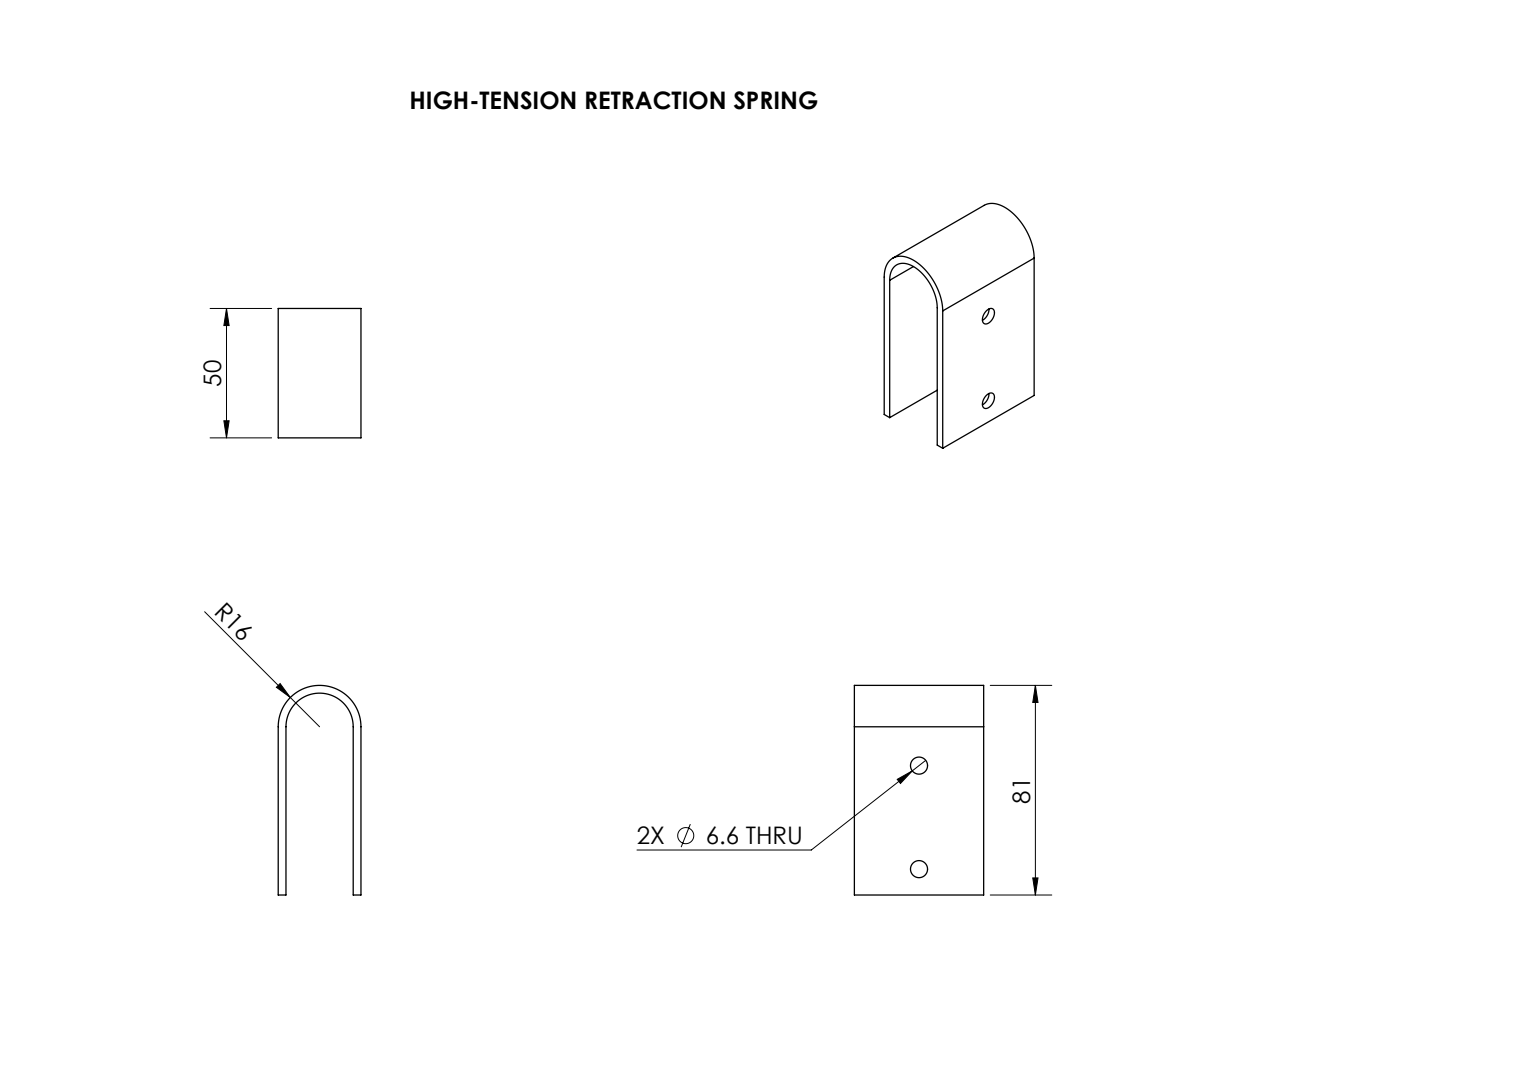
ISO-10303-21;
HEADER;
FILE_DESCRIPTION (('STEP AP214'),
    '1' );
FILE_NAME ('High-Tension Retraction Spring.step',
    '2026-09-24T10:26:00',
    ( '' ),
    ( '' ),
    'SwSTEP 2.0',
    'SolidWorks 2026',
    '' );
FILE_SCHEMA (( 'AUTOMOTIVE_DESIGN' ));
ENDSEC;

DATA;
#71=MECHANICAL_DESIGN_GEOMETRIC_PRESENTATION_REPRESENTATION('',(#7530),#1232);
#73=VERTEX_POINT ( 'NONE', #1987 ) ;
#74=AXIS2_PLACEMENT_3D ( 'NONE', #8274, #12524, #8346 ) ;
#146=ORIENTED_EDGE ( 'NONE', *, *, #7792, .F. ) ;
#147=EDGE_LOOP ( 'NONE', ( #10800, #705, #1394, #14407 ) ) ;
#167=CARTESIAN_POINT ( 'NONE',  ( 0.000000000000000000, 0.000000000000000000, 0.000000000000000000 ) ) ;
#344=ORIENTED_EDGE ( 'NONE', *, *, #679, .T. ) ;
#371=LINE ( 'NONE', #6940, #6098 ) ;
#406=EDGE_LOOP ( 'NONE', ( #12305, #13878, #13303, #2200 ) ) ;
#471=( LENGTH_UNIT ( ) NAMED_UNIT ( * ) SI_UNIT ( .MILLI., .METRE. ) );
#524=VECTOR ( 'NONE', #14360, 1000.000000000000000 ) ;
#530=FACE_BOUND ( 'NONE', #4280, .T. ) ;
#548=PRESENTATION_STYLE_ASSIGNMENT (( #10489 ) ) ;
#575=CARTESIAN_POINT ( 'NONE',  ( 79.68170757442804586, 124.5765550933606249, 25.00000000000000000 ) ) ;
#595=CARTESIAN_POINT ( 'NONE',  ( 79.68170757442804586, 59.57655509336061073, -25.00000000000000000 ) ) ;
#604=ORIENTED_EDGE ( 'NONE', *, *, #5491, .T. ) ;
#619=VERTEX_POINT ( 'NONE', #10072 ) ;
#629=( NAMED_UNIT ( * ) SI_UNIT ( $, .STERADIAN. ) SOLID_ANGLE_UNIT ( ) );
#656=AXIS2_PLACEMENT_3D ( 'NONE', #5018, #7273, #14033 ) ;
#679=EDGE_CURVE ( 'NONE', #13538, #9142, #13956, .T. ) ;
#688=CARTESIAN_POINT ( 'NONE',  ( 92.68170757442806007, 124.5765550933605965, 25.00000000000000000 ) ) ;
#704=VECTOR ( 'NONE', #1188, 1000.000000000000000 ) ;
#705=ORIENTED_EDGE ( 'NONE', *, *, #5491, .F. ) ;
#713=AXIS2_PLACEMENT_3D ( 'NONE', #14232, #7612, #6386 ) ;
#745=CARTESIAN_POINT ( 'NONE',  ( 105.6817075744281311, 124.5765550933606107, 25.00000000000000000 ) ) ;
#749=VECTOR ( 'NONE', #1705, 1000.000000000000000 ) ;
#843=CARTESIAN_POINT ( 'NONE',  ( 76.68170757442798902, 124.5765550933606249, 25.00000000000000000 ) ) ;
#858=DIRECTION ( 'NONE',  ( 1.000000000000000000, 0.000000000000000000, 0.000000000000000000 ) ) ;
#868=EDGE_CURVE ( 'NONE', #3118, #5760, #13014, .T. ) ;
#872=AXIS2_PLACEMENT_3D ( 'NONE', #10007, #2111, #11927 ) ;
#906=DIRECTION ( 'NONE',  ( 0.000000000000000000, 1.000000000000000000, 0.000000000000000000 ) ) ;
#907=CARTESIAN_POINT ( 'NONE',  ( 108.6817075744280174, 69.57655509336049704, 3.300000000000013589 ) ) ;
#929=LINE ( 'NONE', #7732, #11392 ) ;
#970=EDGE_LOOP ( 'NONE', ( #14106, #13551, #3898, #10691 ) ) ;
#985=LINE ( 'NONE', #843, #7180 ) ;
#1177=CIRCLE ( 'NONE', #713, 3.299999999999997158 ) ;
#1188=DIRECTION ( 'NONE',  ( -1.000000000000000000, 0.000000000000000000, 0.000000000000000000 ) ) ;
#1232=( GEOMETRIC_REPRESENTATION_CONTEXT ( 3 ) GLOBAL_UNCERTAINTY_ASSIGNED_CONTEXT ( ( #9384 ) ) GLOBAL_UNIT_ASSIGNED_CONTEXT ( ( #471, #8358, #629 ) ) REPRESENTATION_CONTEXT ( 'NONE', 'WORKASPACE' ) );
#1243=DIRECTION ( 'NONE',  ( -1.000000000000000000, 0.000000000000000000, 0.000000000000000000 ) ) ;
#1298=DIRECTION ( 'NONE',  ( 1.000000000000000000, 0.000000000000000000, 0.000000000000000000 ) ) ;
#1373=AXIS2_PLACEMENT_3D ( 'NONE', #5187, #4969, #7375 ) ;
#1393=VERTEX_POINT ( 'NONE', #9403 ) ;
#1394=ORIENTED_EDGE ( 'NONE', *, *, #679, .F. ) ;
#1475=LINE ( 'NONE', #2572, #5846 ) ;
#1487=ORIENTED_EDGE ( 'NONE', *, *, #12210, .T. ) ;
#1492=CARTESIAN_POINT ( 'NONE',  ( 108.6817075744280174, 109.5765550933605113, 1.102182119232617753E-14 ) ) ;
#1518=FILL_AREA_STYLE ('',( #12707 ) ) ;
#1556=CYLINDRICAL_SURFACE ( 'NONE', #13817, 3.299999999999997158 ) ;
#1558=( NAMED_UNIT ( * ) SI_UNIT ( $, .STERADIAN. ) SOLID_ANGLE_UNIT ( ) );
#1560=DIRECTION ( 'NONE',  ( 0.000000000000000000, 0.000000000000000000, 1.000000000000000000 ) ) ;
#1599=AXIS2_PLACEMENT_3D ( 'NONE', #5171, #7423, #11909 ) ;
#1606=EDGE_CURVE ( 'NONE', #1393, #8011, #1475, .T. ) ;
#1681=DIRECTION ( 'NONE',  ( 0.000000000000000000, 0.000000000000000000, -1.000000000000000000 ) ) ;
#1704=LINE ( 'NONE', #14151, #10227 ) ;
#1705=DIRECTION ( 'NONE',  ( 2.133709875451472726E-16, -1.000000000000000000, -0.000000000000000000 ) ) ;
#1708=VECTOR ( 'NONE', #2266, 1000.000000000000000 ) ;
#1717=SURFACE_STYLE_FILL_AREA ( #13940 ) ;
#1721=AXIS2_PLACEMENT_3D ( 'NONE', #688, #4065, #2281 ) ;
#1773=DIRECTION ( 'NONE',  ( -1.000000000000000000, 0.000000000000000000, 0.000000000000000000 ) ) ;
#1798=LINE ( 'NONE', #11825, #7044 ) ;
#1807=EDGE_LOOP ( 'NONE', ( #11288, #9763, #3211, #9884 ) ) ;
#1871=ADVANCED_FACE ( 'NONE', ( #12299 ), #3099, .F. ) ;
#1888=AXIS2_PLACEMENT_3D ( 'NONE', #7294, #2996, #12863 ) ;
#1979=FACE_OUTER_BOUND ( 'NONE', #5149, .T. ) ;
#1987=CARTESIAN_POINT ( 'NONE',  ( 79.68170757442804586, 59.57655509336061073, 25.00000000000000000 ) ) ;
#1996=LINE ( 'NONE', #12988, #749 ) ;
#2030=EDGE_CURVE ( 'NONE', #619, #2684, #5361, .T. ) ;
#2043=CIRCLE ( 'NONE', #7627, 3.299999999999997158 ) ;
#2050=ORIENTED_EDGE ( 'NONE', *, *, #4383, .F. ) ;
#2111=DIRECTION ( 'NONE',  ( 0.000000000000000000, -1.000000000000000000, 0.000000000000000000 ) ) ;
#2114=DIRECTION ( 'NONE',  ( 0.000000000000000000, 0.000000000000000000, -1.000000000000000000 ) ) ;
#2200=ORIENTED_EDGE ( 'NONE', *, *, #5207, .T. ) ;
#2266=DIRECTION ( 'NONE',  ( 0.000000000000000000, 0.000000000000000000, -1.000000000000000000 ) ) ;
#2281=DIRECTION ( 'NONE',  ( -1.000000000000000000, 0.000000000000000000, 0.000000000000000000 ) ) ;
#2305=PLANE ( 'NONE',  #12341 ) ;
#2311=EDGE_CURVE ( 'NONE', #5760, #13538, #5795, .T. ) ;
#2340=CARTESIAN_POINT ( 'NONE',  ( 92.68170757442806007, 124.5765550933605965, 25.00000000000000000 ) ) ;
#2344=CARTESIAN_POINT ( 'NONE',  ( 108.6817075744280174, 69.57655509336049704, -3.299999999999981171 ) ) ;
#2414=DIRECTION ( 'NONE',  ( -1.000000000000000000, 0.000000000000000000, 0.000000000000000000 ) ) ;
#2515=EDGE_CURVE ( 'NONE', #4441, #2985, #8459, .T. ) ;
#2528=ADVANCED_FACE ( 'NONE', ( #6107 ), #5028, .F. ) ;
#2572=CARTESIAN_POINT ( 'NONE',  ( 76.68170757442798902, 124.5765550933606249, -25.00000000000000000 ) ) ;
#2596=CARTESIAN_POINT ( 'NONE',  ( 108.6817075744280174, 109.5765550933605113, 1.102182119232617753E-14 ) ) ;
#2616=SURFACE_SIDE_STYLE ('',( #5960 ) ) ;
#2636=CARTESIAN_POINT ( 'NONE',  ( 108.6817075744280174, 69.57655509336049704, 1.592040838891559450E-14 ) ) ;
#2650=VECTOR ( 'NONE', #13343, 1000.000000000000000 ) ;
#2684=VERTEX_POINT ( 'NONE', #3272 ) ;
#2701=EDGE_CURVE ( 'NONE', #11645, #2779, #7907, .T. ) ;
#2723=EDGE_CURVE ( 'NONE', #11645, #12380, #9019, .T. ) ;
#2746=CARTESIAN_POINT ( 'NONE',  ( 92.68170757442806007, 124.5765550933605965, 25.00000000000000000 ) ) ;
#2755=DIRECTION ( 'NONE',  ( 1.000000000000000000, 0.000000000000000000, 0.000000000000000000 ) ) ;
#2771=CARTESIAN_POINT ( 'NONE',  ( 105.6817075744280174, 109.5765550933605113, -3.299999999999986500 ) ) ;
#2779=VERTEX_POINT ( 'NONE', #5522 ) ;
#2839=CARTESIAN_POINT ( 'NONE',  ( 76.68170757442798902, 124.5765550933606249, 25.00000000000000000 ) ) ;
#2862=LINE ( 'NONE', #12874, #11439 ) ;
#2912=FACE_OUTER_BOUND ( 'NONE', #9549, .T. ) ;
#2979=DIRECTION ( 'NONE',  ( 0.000000000000000000, 0.000000000000000000, -1.000000000000000000 ) ) ;
#2985=VERTEX_POINT ( 'NONE', #4346 ) ;
#2996=DIRECTION ( 'NONE',  ( 1.000000000000000000, 0.000000000000000000, 0.000000000000000000 ) ) ;
#3003=VERTEX_POINT ( 'NONE', #12232 ) ;
#3020=ORIENTED_EDGE ( 'NONE', *, *, #11613, .T. ) ;
#3022=CARTESIAN_POINT ( 'NONE',  ( 108.6817075744280174, 69.57655509336049704, 3.300000000000013589 ) ) ;
#3071=( GEOMETRIC_REPRESENTATION_CONTEXT ( 3 ) GLOBAL_UNCERTAINTY_ASSIGNED_CONTEXT ( ( #3983 ) ) GLOBAL_UNIT_ASSIGNED_CONTEXT ( ( #11535, #10370, #9264 ) ) REPRESENTATION_CONTEXT ( 'NONE', 'WORKASPACE' ) );
#3090=CARTESIAN_POINT ( 'NONE',  ( 108.6817075744280174, 109.5765550933605113, -3.299999999999986500 ) ) ;
#3096=ORIENTED_EDGE ( 'NONE', *, *, #7792, .T. ) ;
#3099=CYLINDRICAL_SURFACE ( 'NONE', #10041, 3.299999999999997158 ) ;
#3118=VERTEX_POINT ( 'NONE', #5219 ) ;
#3211=ORIENTED_EDGE ( 'NONE', *, *, #868, .F. ) ;
#3214=CARTESIAN_POINT ( 'NONE',  ( 92.68170757442806007, 124.5765550933605965, 25.00000000000000000 ) ) ;
#3253=LINE ( 'NONE', #9903, #5813 ) ;
#3272=CARTESIAN_POINT ( 'NONE',  ( 105.6817075744280174, 69.57655509336049704, -3.299999999999981171 ) ) ;
#3348=DIRECTION ( 'NONE',  ( 0.000000000000000000, -1.000000000000000000, 0.000000000000000000 ) ) ;
#3373=CARTESIAN_POINT ( 'NONE',  ( 108.6817075744280174, 109.5765550933605113, 3.300000000000008260 ) ) ;
#3449=CYLINDRICAL_SURFACE ( 'NONE', #6558, 13.00000000000002487 ) ;
#3453=AXIS2_PLACEMENT_3D ( 'NONE', #9492, #3717, #7286 ) ;
#3528=ORIENTED_EDGE ( 'NONE', *, *, #6801, .T. ) ;
#3559=FACE_OUTER_BOUND ( 'NONE', #406, .T. ) ;
#3597=LINE ( 'NONE', #10235, #4268 ) ;
#3601=EDGE_CURVE ( 'NONE', #619, #13436, #9629, .T. ) ;
#3628=CARTESIAN_POINT ( 'NONE',  ( 108.6817075744280174, 109.5765550933605113, -3.299999999999986500 ) ) ;
#3717=DIRECTION ( 'NONE',  ( 1.000000000000000000, 2.133709875451472726E-16, 0.000000000000000000 ) ) ;
#3736=DIRECTION ( 'NONE',  ( 1.000000000000000000, 0.000000000000000000, 0.000000000000000000 ) ) ;
#3766=DIRECTION ( 'NONE',  ( 1.000000000000000000, 0.000000000000000000, 0.000000000000000000 ) ) ;
#3863=DIRECTION ( 'NONE',  ( 2.133709875451472726E-16, -1.000000000000000000, -0.000000000000000000 ) ) ;
#3872=FACE_OUTER_BOUND ( 'NONE', #8424, .T. ) ;
#3881=DIRECTION ( 'NONE',  ( 0.000000000000000000, 0.000000000000000000, 1.000000000000000000 ) ) ;
#3898=ORIENTED_EDGE ( 'NONE', *, *, #9778, .T. ) ;
#3970=EDGE_CURVE ( 'NONE', #6982, #1393, #11344, .T. ) ;
#3983=UNCERTAINTY_MEASURE_WITH_UNIT (LENGTH_MEASURE( 1.000000000000000082E-05 ), #11535, 'distance_accuracy_value', 'NONE');
#4065=DIRECTION ( 'NONE',  ( 0.000000000000000000, 0.000000000000000000, -1.000000000000000000 ) ) ;
#4164=CARTESIAN_POINT ( 'NONE',  ( 108.6817075744280743, 124.5765550933606107, -25.00000000000000000 ) ) ;
#4252=CARTESIAN_POINT ( 'NONE',  ( 79.68170757442804586, 59.57655509336061073, -25.00000000000000000 ) ) ;
#4268=VECTOR ( 'NONE', #2414, 1000.000000000000000 ) ;
#4280=EDGE_LOOP ( 'NONE', ( #5320, #13667 ) ) ;
#4299=CARTESIAN_POINT ( 'NONE',  ( 108.6817075744280743, 59.57655509336061073, -25.00000000000000000 ) ) ;
#4302=ADVANCED_FACE ( 'NONE', ( #530, #10623, #11866 ), #8414, .T. ) ;
#4346=CARTESIAN_POINT ( 'NONE',  ( 105.6817075744281311, 124.5765550933606107, -25.00000000000000000 ) ) ;
#4371=ORIENTED_EDGE ( 'NONE', *, *, #9778, .F. ) ;
#4383=EDGE_CURVE ( 'NONE', #2684, #619, #4527, .T. ) ;
#4429=VECTOR ( 'NONE', #13663, 1000.000000000000000 ) ;
#4441=VERTEX_POINT ( 'NONE', #8845 ) ;
#4464=AXIS2_PLACEMENT_3D ( 'NONE', #13909, #3881, #8316 ) ;
#4490=LINE ( 'NONE', #2344, #524 ) ;
#4527=CIRCLE ( 'NONE', #9159, 3.299999999999997158 ) ;
#4530=CARTESIAN_POINT ( 'NONE',  ( 108.6817075744280743, 124.5765550933606107, -25.00000000000000000 ) ) ;
#4533=ORIENTED_EDGE ( 'NONE', *, *, #10521, .T. ) ;
#4559=FACE_OUTER_BOUND ( 'NONE', #970, .T. ) ;
#4770=VECTOR ( 'NONE', #3863, 1000.000000000000000 ) ;
#4792=DIRECTION ( 'NONE',  ( 0.000000000000000000, 0.000000000000000000, -1.000000000000000000 ) ) ;
#4847=EDGE_CURVE ( 'NONE', #13538, #1393, #985, .T. ) ;
#4879=CARTESIAN_POINT ( 'NONE',  ( 92.68170757442806007, 124.5765550933605965, -25.00000000000000000 ) ) ;
#4884=ORIENTED_EDGE ( 'NONE', *, *, #6439, .T. ) ;
#4901=ADVANCED_FACE ( 'NONE', ( #11302 ), #2305, .T. ) ;
#4913=DIRECTION ( 'NONE',  ( 0.000000000000000000, 1.000000000000000000, 0.000000000000000000 ) ) ;
#4950=CARTESIAN_POINT ( 'NONE',  ( 105.6817075744281311, 124.5765550933606107, -25.00000000000000000 ) ) ;
#4952=CARTESIAN_POINT ( 'NONE',  ( 105.6817075744281311, 124.5765550933606107, 25.00000000000000000 ) ) ;
#4954=AXIS2_PLACEMENT_3D ( 'NONE', #13901, #12782, #1298 ) ;
#4957=DIRECTION ( 'NONE',  ( 0.000000000000000000, 0.000000000000000000, 1.000000000000000000 ) ) ;
#4959=PLANE ( 'NONE',  #4954 ) ;
#4969=DIRECTION ( 'NONE',  ( -1.000000000000000000, 0.000000000000000000, 0.000000000000000000 ) ) ;
#4976=DIRECTION ( 'NONE',  ( 2.133709875451472726E-16, -1.000000000000000000, -0.000000000000000000 ) ) ;
#5018=CARTESIAN_POINT ( 'NONE',  ( 79.68170757442804586, 124.5765550933606249, 25.00000000000000000 ) ) ;
#5028=PLANE ( 'NONE',  #3453 ) ;
#5132=ORIENTED_EDGE ( 'NONE', *, *, #2515, .T. ) ;
#5138=EDGE_CURVE ( 'NONE', #3118, #14145, #6082, .T. ) ;
#5148=SHAPE_REPRESENTATION_RELATIONSHIP ( 'NONE' , 'NONE' ,  #10940, #5243 ) ;
#5149=EDGE_LOOP ( 'NONE', ( #13973, #11717, #6274, #14396 ) ) ;
#5156=ORIENTED_EDGE ( 'NONE', *, *, #1606, .F. ) ;
#5171=CARTESIAN_POINT ( 'NONE',  ( 105.6817075744280174, 109.5765550933605113, 1.102182119232617753E-14 ) ) ;
#5187=CARTESIAN_POINT ( 'NONE',  ( 105.6817075744280174, 69.57655509336051125, 1.592040838891559450E-14 ) ) ;
#5203=COLOUR_RGB ( '', 0.66274510, 0.83137255, 0.94901961) ;
#5207=EDGE_CURVE ( 'NONE', #12380, #11468, #1177, .T. ) ;
#5219=CARTESIAN_POINT ( 'NONE',  ( 108.6817075744280743, 59.57655509336061073, 25.00000000000000000 ) ) ;
#5243=ADVANCED_BREP_SHAPE_REPRESENTATION ( '', ( #11564, #11025 ), #7056 ) ;
#5273=EDGE_CURVE ( 'NONE', #2779, #11468, #3253, .T. ) ;
#5276=DIRECTION ( 'NONE',  ( -1.000000000000000000, 0.000000000000000000, 0.000000000000000000 ) ) ;
#5277=DIRECTION ( 'NONE',  ( 1.000000000000000000, 0.000000000000000000, 0.000000000000000000 ) ) ;
#5320=ORIENTED_EDGE ( 'NONE', *, *, #2701, .F. ) ;
#5361=CIRCLE ( 'NONE', #1373, 3.299999999999997158 ) ;
#5418=ADVANCED_FACE ( 'NONE', ( #6128 ), #8173, .F. ) ;
#5424=CARTESIAN_POINT ( 'NONE',  ( 79.68170757442804586, 59.57655509336061073, 25.00000000000000000 ) ) ;
#5441=DIRECTION ( 'NONE',  ( 1.000000000000000000, 0.000000000000000000, 0.000000000000000000 ) ) ;
#5491=EDGE_CURVE ( 'NONE', #9142, #8011, #2862, .T. ) ;
#5505=AXIS2_PLACEMENT_3D ( 'NONE', #7465, #10637, #6381 ) ;
#5522=CARTESIAN_POINT ( 'NONE',  ( 105.6817075744280174, 109.5765550933605113, 3.300000000000008260 ) ) ;
#5531=VERTEX_POINT ( 'NONE', #4252 ) ;
#5596=ORIENTED_EDGE ( 'NONE', *, *, #3970, .F. ) ;
#5760=VERTEX_POINT ( 'NONE', #10430 ) ;
#5795=CIRCLE ( 'NONE', #14021, 16.00000000000001421 ) ;
#5813=VECTOR ( 'NONE', #10988, 1000.000000000000000 ) ;
#5833=APPLICATION_CONTEXT ( 'automotive_design' ) ;
#5846=VECTOR ( 'NONE', #6884, 1000.000000000000000 ) ;
#5960=SURFACE_STYLE_FILL_AREA ( #1518 ) ;
#6024=ADVANCED_FACE ( 'NONE', ( #3559 ), #1556, .F. ) ;
#6036=SURFACE_STYLE_USAGE ( .BOTH. , #2616 ) ;
#6063=DIRECTION ( 'NONE',  ( 0.000000000000000000, 0.000000000000000000, 1.000000000000000000 ) ) ;
#6082=LINE ( 'NONE', #7109, #13045 ) ;
#6093=ORIENTED_EDGE ( 'NONE', *, *, #2701, .T. ) ;
#6098=VECTOR ( 'NONE', #4976, 1000.000000000000000 ) ;
#6107=FACE_OUTER_BOUND ( 'NONE', #147, .T. ) ;
#6108=LINE ( 'NONE', #4952, #13540 ) ;
#6128=FACE_OUTER_BOUND ( 'NONE', #6849, .T. ) ;
#6188=DIRECTION ( 'NONE',  ( 1.000000000000000000, 0.000000000000000000, 0.000000000000000000 ) ) ;
#6274=ORIENTED_EDGE ( 'NONE', *, *, #8411, .T. ) ;
#6281=PRODUCT_CONTEXT ( 'NONE', #5833, 'mechanical' ) ;
#6290=ORIENTED_EDGE ( 'NONE', *, *, #2515, .F. ) ;
#6292=CARTESIAN_POINT ( 'NONE',  ( 105.6817075744280174, 69.57655509336051125, 1.592040838891559450E-14 ) ) ;
#6372=ORIENTED_EDGE ( 'NONE', *, *, #13541, .F. ) ;
#6381=DIRECTION ( 'NONE',  ( 1.000000000000000000, 0.000000000000000000, 0.000000000000000000 ) ) ;
#6386=DIRECTION ( 'NONE',  ( 0.000000000000000000, 0.000000000000000000, -1.000000000000000000 ) ) ;
#6423=DIRECTION ( 'NONE',  ( 1.000000000000000000, 0.000000000000000000, 0.000000000000000000 ) ) ;
#6439=EDGE_CURVE ( 'NONE', #5531, #8011, #9354, .T. ) ;
#6452=ORIENTED_EDGE ( 'NONE', *, *, #12896, .T. ) ;
#6454=ADVANCED_FACE ( 'NONE', ( #10112 ), #9004, .F. ) ;
#6505=CIRCLE ( 'NONE', #12129, 3.299999999999997158 ) ;
#6524=DIRECTION ( 'NONE',  ( 0.000000000000000000, 0.000000000000000000, 1.000000000000000000 ) ) ;
#6558=AXIS2_PLACEMENT_3D ( 'NONE', #2340, #11267, #1243 ) ;
#6653=ORIENTED_EDGE ( 'NONE', *, *, #5207, .F. ) ;
#6766=EDGE_LOOP ( 'NONE', ( #6653, #9405 ) ) ;
#6783=CIRCLE ( 'NONE', #1888, 3.299999999999997158 ) ;
#6801=EDGE_CURVE ( 'NONE', #3003, #2985, #6108, .T. ) ;
#6829=PRODUCT_DEFINITION_SHAPE ( 'NONE', 'NONE',  #11417 ) ;
#6849=EDGE_LOOP ( 'NONE', ( #5156, #5596, #7420, #11471, #5132, #4533, #1487, #4884 ) ) ;
#6865=EDGE_CURVE ( 'NONE', #14145, #6982, #10665, .T. ) ;
#6884=DIRECTION ( 'NONE',  ( 2.133709875451472726E-16, -1.000000000000000000, -0.000000000000000000 ) ) ;
#6940=CARTESIAN_POINT ( 'NONE',  ( 79.68170757442804586, 124.5765550933606249, -25.00000000000000000 ) ) ;
#6959=VECTOR ( 'NONE', #9710, 1000.000000000000000 ) ;
#6982=VERTEX_POINT ( 'NONE', #4530 ) ;
#7044=VECTOR ( 'NONE', #2979, 1000.000000000000000 ) ;
#7056=( GEOMETRIC_REPRESENTATION_CONTEXT ( 3 ) GLOBAL_UNCERTAINTY_ASSIGNED_CONTEXT ( ( #9235 ) ) GLOBAL_UNIT_ASSIGNED_CONTEXT ( ( #11658, #9469, #1558 ) ) REPRESENTATION_CONTEXT ( 'NONE', 'WORKASPACE' ) );
#7062=PRESENTATION_STYLE_ASSIGNMENT (( #6036 ) ) ;
#7086=CARTESIAN_POINT ( 'NONE',  ( 105.6817075744280743, 59.57655509336061073, 25.00000000000000000 ) ) ;
#7091=VECTOR ( 'NONE', #906, 1000.000000000000000 ) ;
#7109=CARTESIAN_POINT ( 'NONE',  ( 108.6817075744280743, 59.57655509336061073, 25.00000000000000000 ) ) ;
#7110=SURFACE_SIDE_STYLE ('',( #1717 ) ) ;
#7180=VECTOR ( 'NONE', #7565, 1000.000000000000000 ) ;
#7205=EDGE_CURVE ( 'NONE', #11468, #12380, #10697, .T. ) ;
#7228=CARTESIAN_POINT ( 'NONE',  ( 79.68170757442804586, 124.5765550933606249, 25.00000000000000000 ) ) ;
#7242=EDGE_CURVE ( 'NONE', #2779, #11645, #6505, .T. ) ;
#7273=DIRECTION ( 'NONE',  ( 1.000000000000000000, 2.133709875451472726E-16, 0.000000000000000000 ) ) ;
#7286=DIRECTION ( 'NONE',  ( -2.133709875451472726E-16, 1.000000000000000000, 0.000000000000000000 ) ) ;
#7294=CARTESIAN_POINT ( 'NONE',  ( 108.6817075744280174, 69.57655509336049704, 1.592040838891559450E-14 ) ) ;
#7326=PRODUCT_DEFINITION_FORMATION_WITH_SPECIFIED_SOURCE ( 'ANY', '', #12672, .NOT_KNOWN. ) ;
#7375=DIRECTION ( 'NONE',  ( 0.000000000000000000, 0.000000000000000000, 1.000000000000000000 ) ) ;
#7420=ORIENTED_EDGE ( 'NONE', *, *, #6865, .F. ) ;
#7423=DIRECTION ( 'NONE',  ( -1.000000000000000000, 0.000000000000000000, 0.000000000000000000 ) ) ;
#7465=CARTESIAN_POINT ( 'NONE',  ( 92.68170757442806007, 124.5765550933605965, -25.00000000000000000 ) ) ;
#7487=EDGE_LOOP ( 'NONE', ( #6290, #11515, #3096, #3528 ) ) ;
#7529=DIRECTION ( 'NONE',  ( 0.000000000000000000, 0.000000000000000000, -1.000000000000000000 ) ) ;
#7530=STYLED_ITEM ( 'NONE', ( #548 ), #5243 ) ;
#7565=DIRECTION ( 'NONE',  ( 0.000000000000000000, 0.000000000000000000, -1.000000000000000000 ) ) ;
#7588=EDGE_LOOP ( 'NONE', ( #9699, #12550, #14101, #3020 ) ) ;
#7593=AXIS2_PLACEMENT_3D ( 'NONE', #745, #1773, #6063 ) ;
#7612=DIRECTION ( 'NONE',  ( 1.000000000000000000, 0.000000000000000000, 0.000000000000000000 ) ) ;
#7627=AXIS2_PLACEMENT_3D ( 'NONE', #13732, #2755, #13671 ) ;
#7646=DIRECTION ( 'NONE',  ( 0.000000000000000000, 0.000000000000000000, 1.000000000000000000 ) ) ;
#7651=CIRCLE ( 'NONE', #9777, 13.00000000000002487 ) ;
#7664=ORIENTED_EDGE ( 'NONE', *, *, #9005, .T. ) ;
#7732=CARTESIAN_POINT ( 'NONE',  ( 108.6817075744280743, 124.5765550933606107, 25.00000000000000000 ) ) ;
#7734=CARTESIAN_POINT ( 'NONE',  ( 108.6817075744280174, 69.57655509336049704, 1.592040838891559450E-14 ) ) ;
#7739=CARTESIAN_POINT ( 'NONE',  ( 76.68170757442798902, 124.5765550933606249, 25.00000000000000000 ) ) ;
#7782=ORIENTED_EDGE ( 'NONE', *, *, #2723, .F. ) ;
#7786=DIRECTION ( 'NONE',  ( 0.000000000000000000, 0.000000000000000000, -1.000000000000000000 ) ) ;
#7792=EDGE_CURVE ( 'NONE', #13250, #3003, #1704, .T. ) ;
#7823=APPLICATION_CONTEXT ( 'automotive_design' ) ;
#7907=CIRCLE ( 'NONE', #1599, 3.299999999999997158 ) ;
#7932=CARTESIAN_POINT ( 'NONE',  ( 105.6817075744280174, 109.5765550933605113, 1.102182119232617753E-14 ) ) ;
#7994=DIRECTION ( 'NONE',  ( 1.000000000000000000, 0.000000000000000000, 0.000000000000000000 ) ) ;
#8011=VERTEX_POINT ( 'NONE', #13341 ) ;
#8132=DIRECTION ( 'NONE',  ( 0.000000000000000000, 0.000000000000000000, -1.000000000000000000 ) ) ;
#8173=PLANE ( 'NONE',  #4464 ) ;
#8274=CARTESIAN_POINT ( 'NONE',  ( 108.6817075744280743, 124.5765550933606107, 25.00000000000000000 ) ) ;
#8316=DIRECTION ( 'NONE',  ( 1.000000000000000000, 0.000000000000000000, 0.000000000000000000 ) ) ;
#8346=DIRECTION ( 'NONE',  ( 0.000000000000000000, 0.000000000000000000, 1.000000000000000000 ) ) ;
#8358=( NAMED_UNIT ( * ) PLANE_ANGLE_UNIT ( ) SI_UNIT ( $, .RADIAN. ) );
#8369=CARTESIAN_POINT ( 'NONE',  ( 108.6817075744280174, 69.57655509336049704, -3.299999999999981171 ) ) ;
#8411=EDGE_CURVE ( 'NONE', #13436, #8560, #2043, .T. ) ;
#8414=PLANE ( 'NONE',  #7593 ) ;
#8424=EDGE_LOOP ( 'NONE', ( #344, #10206, #12578, #4371, #146, #9198, #13128, #9967 ) ) ;
#8459=LINE ( 'NONE', #4950, #10207 ) ;
#8505=CARTESIAN_POINT ( 'NONE',  ( 108.6817075744280743, 59.57655509336061073, -25.00000000000000000 ) ) ;
#8523=LINE ( 'NONE', #4299, #8703 ) ;
#8560=VERTEX_POINT ( 'NONE', #8369 ) ;
#8604=ADVANCED_FACE ( 'NONE', ( #2912 ), #9556, .T. ) ;
#8607=VECTOR ( 'NONE', #12624, 1000.000000000000000 ) ;
#8662=DIRECTION ( 'NONE',  ( -1.000000000000000000, 0.000000000000000000, 0.000000000000000000 ) ) ;
#8703=VECTOR ( 'NONE', #8662, 1000.000000000000000 ) ;
#8845=CARTESIAN_POINT ( 'NONE',  ( 105.6817075744280743, 59.57655509336061073, -25.00000000000000000 ) ) ;
#8856=LINE ( 'NONE', #5424, #2650 ) ;
#8858=AXIS2_PLACEMENT_3D ( 'NONE', #2636, #3736, #1681 ) ;
#8990=ADVANCED_FACE ( 'NONE', ( #9724 ), #14199, .T. ) ;
#9004=CYLINDRICAL_SURFACE ( 'NONE', #8858, 3.299999999999997158 ) ;
#9005=EDGE_CURVE ( 'NONE', #5760, #6982, #929, .T. ) ;
#9019=LINE ( 'NONE', #3628, #4429 ) ;
#9086=ORIENTED_EDGE ( 'NONE', *, *, #5273, .T. ) ;
#9092=CARTESIAN_POINT ( 'NONE',  ( 79.68170757442804586, 59.57655509336061073, 25.00000000000000000 ) ) ;
#9142=VERTEX_POINT ( 'NONE', #11249 ) ;
#9159=AXIS2_PLACEMENT_3D ( 'NONE', #6292, #5276, #10694 ) ;
#9198=ORIENTED_EDGE ( 'NONE', *, *, #10840, .F. ) ;
#9235=UNCERTAINTY_MEASURE_WITH_UNIT (LENGTH_MEASURE( 1.000000000000000082E-05 ), #11658, 'distance_accuracy_value', 'NONE');
#9246=ORIENTED_EDGE ( 'NONE', *, *, #12210, .F. ) ;
#9264=( NAMED_UNIT ( * ) SI_UNIT ( $, .STERADIAN. ) SOLID_ANGLE_UNIT ( ) );
#9308=FACE_BOUND ( 'NONE', #12962, .T. ) ;
#9309=EDGE_CURVE ( 'NONE', #11268, #13323, #12706, .T. ) ;
#9354=LINE ( 'NONE', #595, #704 ) ;
#9384=UNCERTAINTY_MEASURE_WITH_UNIT (LENGTH_MEASURE( 1.000000000000000082E-05 ), #471, 'distance_accuracy_value', 'NONE');
#9403=CARTESIAN_POINT ( 'NONE',  ( 76.68170757442798902, 124.5765550933606249, -25.00000000000000000 ) ) ;
#9405=ORIENTED_EDGE ( 'NONE', *, *, #7205, .F. ) ;
#9416=DIRECTION ( 'NONE',  ( 0.000000000000000000, 0.000000000000000000, -1.000000000000000000 ) ) ;
#9469=( NAMED_UNIT ( * ) PLANE_ANGLE_UNIT ( ) SI_UNIT ( $, .RADIAN. ) );
#9492=CARTESIAN_POINT ( 'NONE',  ( 76.68170757442798902, 124.5765550933606249, 25.00000000000000000 ) ) ;
#9549=EDGE_LOOP ( 'NONE', ( #9246, #13391, #6452, #13924 ) ) ;
#9556=PLANE ( 'NONE',  #656 ) ;
#9600=CIRCLE ( 'NONE', #11463, 13.00000000000002487 ) ;
#9629=LINE ( 'NONE', #907, #14311 ) ;
#9682=ORIENTED_EDGE ( 'NONE', *, *, #5138, .F. ) ;
#9699=ORIENTED_EDGE ( 'NONE', *, *, #3601, .F. ) ;
#9710=DIRECTION ( 'NONE',  ( 0.000000000000000000, 1.000000000000000000, 0.000000000000000000 ) ) ;
#9724=FACE_OUTER_BOUND ( 'NONE', #9999, .T. ) ;
#9763=ORIENTED_EDGE ( 'NONE', *, *, #9005, .F. ) ;
#9777=AXIS2_PLACEMENT_3D ( 'NONE', #2746, #1560, #3766 ) ;
#9778=EDGE_CURVE ( 'NONE', #3003, #11268, #7651, .T. ) ;
#9858=EDGE_LOOP ( 'NONE', ( #11043, #6372, #11589, #604 ) ) ;
#9884=ORIENTED_EDGE ( 'NONE', *, *, #5138, .T. ) ;
#9903=CARTESIAN_POINT ( 'NONE',  ( 108.6817075744280174, 109.5765550933605113, 3.300000000000008260 ) ) ;
#9907=EDGE_LOOP ( 'NONE', ( #6093, #9086, #13776, #7782 ) ) ;
#9967=ORIENTED_EDGE ( 'NONE', *, *, #2311, .T. ) ;
#9999=EDGE_LOOP ( 'NONE', ( #14114, #9682, #13602, #11045 ) ) ;
#10007=CARTESIAN_POINT ( 'NONE',  ( 108.6817075744280743, 59.57655509336061073, 25.00000000000000000 ) ) ;
#10013=LINE ( 'NONE', #12075, #1708 ) ;
#10041=AXIS2_PLACEMENT_3D ( 'NONE', #12228, #5277, #7529 ) ;
#10072=CARTESIAN_POINT ( 'NONE',  ( 105.6817075744280174, 69.57655509336049704, 3.300000000000013589 ) ) ;
#10088=AXIS2_PLACEMENT_3D ( 'NONE', #7734, #6423, #2114 ) ;
#10112=FACE_OUTER_BOUND ( 'NONE', #7588, .T. ) ;
#10206=ORIENTED_EDGE ( 'NONE', *, *, #14204, .F. ) ;
#10207=VECTOR ( 'NONE', #12859, 1000.000000000000000 ) ;
#10218=ADVANCED_FACE ( 'NONE', ( #1979 ), #12136, .F. ) ;
#10227=VECTOR ( 'NONE', #4913, 1000.000000000000000 ) ;
#10235=CARTESIAN_POINT ( 'NONE',  ( 108.6817075744280743, 59.57655509336061073, 25.00000000000000000 ) ) ;
#10252=ORIENTED_EDGE ( 'NONE', *, *, #4847, .F. ) ;
#10270=DIRECTION ( 'NONE',  ( 0.000000000000000000, 0.000000000000000000, 1.000000000000000000 ) ) ;
#10370=( NAMED_UNIT ( * ) PLANE_ANGLE_UNIT ( ) SI_UNIT ( $, .RADIAN. ) );
#10430=CARTESIAN_POINT ( 'NONE',  ( 108.6817075744280743, 124.5765550933606107, 25.00000000000000000 ) ) ;
#10435=DIRECTION ( 'NONE',  ( 1.000000000000000000, 0.000000000000000000, 0.000000000000000000 ) ) ;
#10489=SURFACE_STYLE_USAGE ( .BOTH. , #7110 ) ;
#10496=DIRECTION ( 'NONE',  ( 1.000000000000000000, 0.000000000000000000, 0.000000000000000000 ) ) ;
#10521=EDGE_CURVE ( 'NONE', #2985, #13323, #9600, .T. ) ;
#10564=DIRECTION ( 'NONE',  ( 0.000000000000000000, 0.000000000000000000, -1.000000000000000000 ) ) ;
#10623=FACE_BOUND ( 'NONE', #13001, .T. ) ;
#10637=DIRECTION ( 'NONE',  ( 0.000000000000000000, 0.000000000000000000, 1.000000000000000000 ) ) ;
#10665=LINE ( 'NONE', #4164, #6959 ) ;
#10691=ORIENTED_EDGE ( 'NONE', *, *, #9309, .T. ) ;
#10694=DIRECTION ( 'NONE',  ( 0.000000000000000000, 0.000000000000000000, 1.000000000000000000 ) ) ;
#10697=CIRCLE ( 'NONE', #13278, 3.299999999999997158 ) ;
#10703=CYLINDRICAL_SURFACE ( 'NONE', #1721, 16.00000000000001421 ) ;
#10800=ORIENTED_EDGE ( 'NONE', *, *, #1606, .T. ) ;
#10825=DIRECTION ( 'NONE',  ( 0.000000000000000000, 0.000000000000000000, -1.000000000000000000 ) ) ;
#10840=EDGE_CURVE ( 'NONE', #3118, #13250, #3597, .T. ) ;
#10910=ADVANCED_FACE ( 'NONE', ( #4559 ), #3449, .F. ) ;
#10940=SHAPE_REPRESENTATION ( 'High-Tension Retraction Spring', ( #11025 ), #7056 ) ;
#10988=DIRECTION ( 'NONE',  ( 1.000000000000000000, 0.000000000000000000, 0.000000000000000000 ) ) ;
#10992=COLOUR_RGB ( '', 0.66274510, 0.83137255, 0.94901961) ;
#11025=AXIS2_PLACEMENT_3D ( 'NONE', #167, #6524, #5441 ) ;
#11042=ORIENTED_EDGE ( 'NONE', *, *, #2030, .F. ) ;
#11043=ORIENTED_EDGE ( 'NONE', *, *, #6439, .F. ) ;
#11045=ORIENTED_EDGE ( 'NONE', *, *, #14400, .T. ) ;
#11134=PRODUCT_DEFINITION_CONTEXT ( 'detailed design', #7823, 'design' ) ;
#11231=ORIENTED_EDGE ( 'NONE', *, *, #11613, .F. ) ;
#11249=CARTESIAN_POINT ( 'NONE',  ( 76.68170757442804586, 59.57655509336061073, 25.00000000000000000 ) ) ;
#11267=DIRECTION ( 'NONE',  ( 0.000000000000000000, 0.000000000000000000, -1.000000000000000000 ) ) ;
#11268=VERTEX_POINT ( 'NONE', #7228 ) ;
#11288=ORIENTED_EDGE ( 'NONE', *, *, #6865, .T. ) ;
#11296=ORIENTED_EDGE ( 'NONE', *, *, #8411, .F. ) ;
#11302=FACE_OUTER_BOUND ( 'NONE', #9858, .T. ) ;
#11344=CIRCLE ( 'NONE', #5505, 16.00000000000001421 ) ;
#11392=VECTOR ( 'NONE', #14340, 1000.000000000000000 ) ;
#11417=PRODUCT_DEFINITION ( 'UNKNOWN', '', #7326, #11134 ) ;
#11439=VECTOR ( 'NONE', #10825, 1000.000000000000000 ) ;
#11463=AXIS2_PLACEMENT_3D ( 'NONE', #4879, #4957, #10435 ) ;
#11468=VERTEX_POINT ( 'NONE', #3373 ) ;
#11471=ORIENTED_EDGE ( 'NONE', *, *, #14435, .T. ) ;
#11501=FACE_OUTER_BOUND ( 'NONE', #1807, .T. ) ;
#11515=ORIENTED_EDGE ( 'NONE', *, *, #14400, .F. ) ;
#11535=( LENGTH_UNIT ( ) NAMED_UNIT ( * ) SI_UNIT ( .MILLI., .METRE. ) );
#11557=CLOSED_SHELL ( 'NONE', ( #1871, #10218, #13952, #2528, #4901, #8604, #10910, #4302, #8990, #14167, #12575, #5418, #6454, #6024 ) ) ;
#11564=MANIFOLD_SOLID_BREP ( 'M6 Clearance Hole1', #11557 ) ;
#11589=ORIENTED_EDGE ( 'NONE', *, *, #14204, .T. ) ;
#11613=EDGE_CURVE ( 'NONE', #8560, #13436, #6783, .T. ) ;
#11645=VERTEX_POINT ( 'NONE', #2771 ) ;
#11658=( LENGTH_UNIT ( ) NAMED_UNIT ( * ) SI_UNIT ( .MILLI., .METRE. ) );
#11717=ORIENTED_EDGE ( 'NONE', *, *, #3601, .T. ) ;
#11815=FILL_AREA_STYLE_COLOUR ( '', #5203 ) ;
#11825=CARTESIAN_POINT ( 'NONE',  ( 105.6817075744280743, 59.57655509336061073, 25.00000000000000000 ) ) ;
#11866=FACE_OUTER_BOUND ( 'NONE', #7487, .T. ) ;
#11909=DIRECTION ( 'NONE',  ( 0.000000000000000000, 0.000000000000000000, 1.000000000000000000 ) ) ;
#11927=DIRECTION ( 'NONE',  ( 0.000000000000000000, 0.000000000000000000, -1.000000000000000000 ) ) ;
#12045=CARTESIAN_POINT ( 'NONE',  ( 108.6817075744280743, 124.5765550933606107, 25.00000000000000000 ) ) ;
#12075=CARTESIAN_POINT ( 'NONE',  ( 79.68170757442804586, 59.57655509336061073, 25.00000000000000000 ) ) ;
#12129=AXIS2_PLACEMENT_3D ( 'NONE', #7932, #12409, #10270 ) ;
#12136=CYLINDRICAL_SURFACE ( 'NONE', #10088, 3.299999999999997158 ) ;
#12210=EDGE_CURVE ( 'NONE', #13323, #5531, #371, .T. ) ;
#12228=CARTESIAN_POINT ( 'NONE',  ( 108.6817075744280174, 109.5765550933605113, 1.102182119232617753E-14 ) ) ;
#12232=CARTESIAN_POINT ( 'NONE',  ( 105.6817075744281311, 124.5765550933606107, 25.00000000000000000 ) ) ;
#12299=FACE_OUTER_BOUND ( 'NONE', #9907, .T. ) ;
#12305=ORIENTED_EDGE ( 'NONE', *, *, #5273, .F. ) ;
#12341=AXIS2_PLACEMENT_3D ( 'NONE', #9092, #3348, #7786 ) ;
#12380=VERTEX_POINT ( 'NONE', #3090 ) ;
#12409=DIRECTION ( 'NONE',  ( -1.000000000000000000, 0.000000000000000000, 0.000000000000000000 ) ) ;
#12524=DIRECTION ( 'NONE',  ( -1.000000000000000000, 0.000000000000000000, 0.000000000000000000 ) ) ;
#12550=ORIENTED_EDGE ( 'NONE', *, *, #2030, .T. ) ;
#12575=ADVANCED_FACE ( 'NONE', ( #3872 ), #4959, .T. ) ;
#12578=ORIENTED_EDGE ( 'NONE', *, *, #12896, .F. ) ;
#12624=DIRECTION ( 'NONE',  ( 0.000000000000000000, 0.000000000000000000, -1.000000000000000000 ) ) ;
#12672=PRODUCT ( 'High-Tension Retraction Spring', 'High-Tension Retraction Spring', '', ( #6281 ) ) ;
#12706=LINE ( 'NONE', #575, #8607 ) ;
#12707=FILL_AREA_STYLE_COLOUR ( '', #10992 ) ;
#12749=EDGE_CURVE ( 'NONE', #2684, #8560, #4490, .T. ) ;
#12782=DIRECTION ( 'NONE',  ( 0.000000000000000000, 0.000000000000000000, 1.000000000000000000 ) ) ;
#12829=PLANE ( 'NONE',  #74 ) ;
#12859=DIRECTION ( 'NONE',  ( 0.000000000000000000, 1.000000000000000000, 0.000000000000000000 ) ) ;
#12863=DIRECTION ( 'NONE',  ( 0.000000000000000000, 0.000000000000000000, -1.000000000000000000 ) ) ;
#12874=CARTESIAN_POINT ( 'NONE',  ( 76.68170757442804586, 59.57655509336061073, 25.00000000000000000 ) ) ;
#12880=MECHANICAL_DESIGN_GEOMETRIC_PRESENTATION_REPRESENTATION('',(#13344),#3071);
#12896=EDGE_CURVE ( 'NONE', #11268, #73, #1996, .T. ) ;
#12962=EDGE_LOOP ( 'NONE', ( #11231, #11296 ) ) ;
#12988=CARTESIAN_POINT ( 'NONE',  ( 79.68170757442804586, 124.5765550933606249, 25.00000000000000000 ) ) ;
#13001=EDGE_LOOP ( 'NONE', ( #2050, #11042 ) ) ;
#13014=LINE ( 'NONE', #12045, #7091 ) ;
#13045=VECTOR ( 'NONE', #10564, 1000.000000000000000 ) ;
#13128=ORIENTED_EDGE ( 'NONE', *, *, #868, .T. ) ;
#13250=VERTEX_POINT ( 'NONE', #7086 ) ;
#13278=AXIS2_PLACEMENT_3D ( 'NONE', #2596, #10496, #4792 ) ;
#13303=ORIENTED_EDGE ( 'NONE', *, *, #2723, .T. ) ;
#13323=VERTEX_POINT ( 'NONE', #13559 ) ;
#13341=CARTESIAN_POINT ( 'NONE',  ( 76.68170757442804586, 59.57655509336061073, -25.00000000000000000 ) ) ;
#13343=DIRECTION ( 'NONE',  ( -1.000000000000000000, 0.000000000000000000, 0.000000000000000000 ) ) ;
#13344=STYLED_ITEM ( 'NONE', ( #7062 ), #11564 ) ;
#13391=ORIENTED_EDGE ( 'NONE', *, *, #9309, .F. ) ;
#13436=VERTEX_POINT ( 'NONE', #3022 ) ;
#13538=VERTEX_POINT ( 'NONE', #7739 ) ;
#13540=VECTOR ( 'NONE', #9416, 1000.000000000000000 ) ;
#13541=EDGE_CURVE ( 'NONE', #73, #5531, #10013, .T. ) ;
#13551=ORIENTED_EDGE ( 'NONE', *, *, #6801, .F. ) ;
#13559=CARTESIAN_POINT ( 'NONE',  ( 79.68170757442804586, 124.5765550933606249, -25.00000000000000000 ) ) ;
#13602=ORIENTED_EDGE ( 'NONE', *, *, #10840, .T. ) ;
#13648=ORIENTED_EDGE ( 'NONE', *, *, #2311, .F. ) ;
#13652=ORIENTED_EDGE ( 'NONE', *, *, #3970, .T. ) ;
#13663=DIRECTION ( 'NONE',  ( 1.000000000000000000, 0.000000000000000000, 0.000000000000000000 ) ) ;
#13667=ORIENTED_EDGE ( 'NONE', *, *, #7242, .F. ) ;
#13671=DIRECTION ( 'NONE',  ( 0.000000000000000000, 0.000000000000000000, -1.000000000000000000 ) ) ;
#13732=CARTESIAN_POINT ( 'NONE',  ( 108.6817075744280174, 69.57655509336049704, 1.592040838891559450E-14 ) ) ;
#13776=ORIENTED_EDGE ( 'NONE', *, *, #7205, .T. ) ;
#13817=AXIS2_PLACEMENT_3D ( 'NONE', #1492, #7994, #8132 ) ;
#13878=ORIENTED_EDGE ( 'NONE', *, *, #7242, .T. ) ;
#13901=CARTESIAN_POINT ( 'NONE',  ( 92.68170757442806007, 124.5765550933605965, 25.00000000000000000 ) ) ;
#13909=CARTESIAN_POINT ( 'NONE',  ( 92.68170757442806007, 124.5765550933605965, -25.00000000000000000 ) ) ;
#13924=ORIENTED_EDGE ( 'NONE', *, *, #13541, .T. ) ;
#13932=FACE_BOUND ( 'NONE', #6766, .T. ) ;
#13940=FILL_AREA_STYLE ('',( #11815 ) ) ;
#13952=ADVANCED_FACE ( 'NONE', ( #13932, #11501, #9308 ), #12829, .F. ) ;
#13956=LINE ( 'NONE', #2839, #4770 ) ;
#13973=ORIENTED_EDGE ( 'NONE', *, *, #4383, .T. ) ;
#14021=AXIS2_PLACEMENT_3D ( 'NONE', #3214, #7646, #858 ) ;
#14033=DIRECTION ( 'NONE',  ( -2.133709875451472726E-16, 1.000000000000000000, 0.000000000000000000 ) ) ;
#14085=FACE_OUTER_BOUND ( 'NONE', #14330, .T. ) ;
#14101=ORIENTED_EDGE ( 'NONE', *, *, #12749, .T. ) ;
#14106=ORIENTED_EDGE ( 'NONE', *, *, #10521, .F. ) ;
#14114=ORIENTED_EDGE ( 'NONE', *, *, #14435, .F. ) ;
#14145=VERTEX_POINT ( 'NONE', #8505 ) ;
#14151=CARTESIAN_POINT ( 'NONE',  ( 105.6817075744281311, 124.5765550933606107, 25.00000000000000000 ) ) ;
#14167=ADVANCED_FACE ( 'NONE', ( #14085 ), #10703, .T. ) ;
#14199=PLANE ( 'NONE',  #872 ) ;
#14202=SHAPE_DEFINITION_REPRESENTATION ( #6829, #10940 ) ;
#14204=EDGE_CURVE ( 'NONE', #73, #9142, #8856, .T. ) ;
#14232=CARTESIAN_POINT ( 'NONE',  ( 108.6817075744280174, 109.5765550933605113, 1.102182119232617753E-14 ) ) ;
#14311=VECTOR ( 'NONE', #6188, 1000.000000000000000 ) ;
#14330=EDGE_LOOP ( 'NONE', ( #13652, #10252, #13648, #7664 ) ) ;
#14340=DIRECTION ( 'NONE',  ( 0.000000000000000000, 0.000000000000000000, -1.000000000000000000 ) ) ;
#14360=DIRECTION ( 'NONE',  ( 1.000000000000000000, 0.000000000000000000, 0.000000000000000000 ) ) ;
#14396=ORIENTED_EDGE ( 'NONE', *, *, #12749, .F. ) ;
#14400=EDGE_CURVE ( 'NONE', #13250, #4441, #1798, .T. ) ;
#14407=ORIENTED_EDGE ( 'NONE', *, *, #4847, .T. ) ;
#14435=EDGE_CURVE ( 'NONE', #14145, #4441, #8523, .T. ) ;
ENDSEC;
END-ISO-10303-21;
